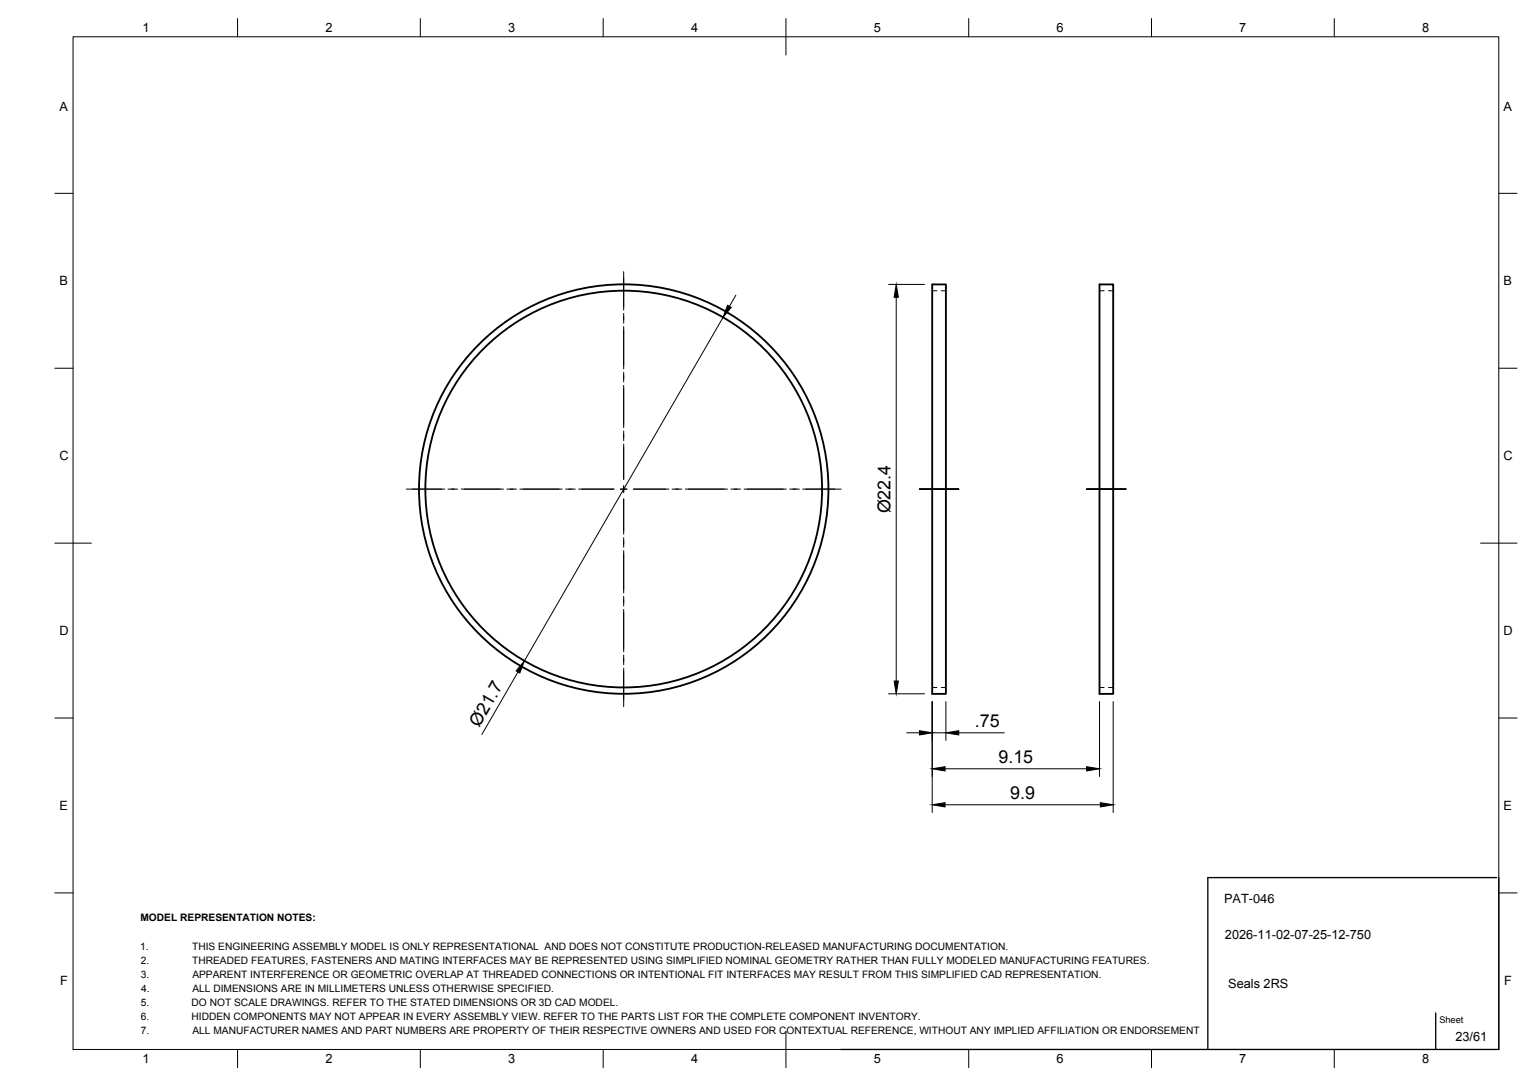
ISO-10303-21;
HEADER;
/* Generated by software containing ST-Developer
 * from STEP Tools, Inc. (www.steptools.com) 
 */

FILE_DESCRIPTION(
/* description */ ('Gear mesh backlash fixture'),
/* implementation_level */ '2;1');

FILE_NAME(
/* name */ 'Seals 2RS.step',
/* time_stamp */ '2026-10-28T03:26:00-07:00',
/* author */ (''),
/* organization */ (''),
/* preprocessor_version */ 'ST-DEVELOPER v20.2',
/* originating_system */ 'Autodesk Translation Framework v15.17.0.0',
/* authorisation */ '');

FILE_SCHEMA (('AUTOMOTIVE_DESIGN { 1 0 10303 214 3 1 1 }'));
ENDSEC;

DATA;
#10=MECHANICAL_DESIGN_GEOMETRIC_PRESENTATION_REPRESENTATION('',(#1038,#1039),#57900);
#932=SHAPE_REPRESENTATION_RELATIONSHIP('SRR','None',#58128,#982);
#982=ADVANCED_BREP_SHAPE_REPRESENTATION('',(#1103,#1104),#57861);
#1038=STYLED_ITEM('',(#58465),#1103);
#1039=STYLED_ITEM('',(#58465),#1104);
#1103=MANIFOLD_SOLID_BREP('Body1',#13598);
#1104=MANIFOLD_SOLID_BREP('Body2',#13599);
#1222=FACE_BOUND('',#2725,.T.);
#1223=FACE_BOUND('',#2728,.T.);
#1224=FACE_BOUND('',#2731,.T.);
#1225=FACE_BOUND('',#2734,.T.);
#1425=PLANE('',#14603);
#1426=PLANE('',#14608);
#1427=PLANE('',#14611);
#1428=PLANE('',#14616);
#1880=FACE_OUTER_BOUND('',#2724,.T.);
#1881=FACE_OUTER_BOUND('',#2726,.T.);
#1882=FACE_OUTER_BOUND('',#2727,.T.);
#1883=FACE_OUTER_BOUND('',#2729,.T.);
#1884=FACE_OUTER_BOUND('',#2730,.T.);
#1885=FACE_OUTER_BOUND('',#2732,.T.);
#1886=FACE_OUTER_BOUND('',#2733,.T.);
#1887=FACE_OUTER_BOUND('',#2735,.T.);
#2724=EDGE_LOOP('',(#9721));
#2725=EDGE_LOOP('',(#9722));
#2726=EDGE_LOOP('',(#9723,#9724,#9725,#9726));
#2727=EDGE_LOOP('',(#9727));
#2728=EDGE_LOOP('',(#9728));
#2729=EDGE_LOOP('',(#9729,#9730,#9731,#9732));
#2730=EDGE_LOOP('',(#9733));
#2731=EDGE_LOOP('',(#9734));
#2732=EDGE_LOOP('',(#9735,#9736,#9737,#9738));
#2733=EDGE_LOOP('',(#9739));
#2734=EDGE_LOOP('',(#9740));
#2735=EDGE_LOOP('',(#9741,#9742,#9743,#9744));
#3609=LINE('',#20541,#4498);
#3610=LINE('',#20546,#4499);
#3611=LINE('',#20555,#4500);
#3612=LINE('',#20560,#4501);
#4498=VECTOR('',#16602,1.119765);
#4499=VECTOR('',#16609,1.085235);
#4500=VECTOR('',#16620,1.119765);
#4501=VECTOR('',#16627,1.085235);
#5391=CIRCLE('',#14604,1.119765);
#5392=CIRCLE('',#14605,1.085235);
#5393=CIRCLE('',#14607,1.119765);
#5394=CIRCLE('',#14609,1.085235);
#5395=CIRCLE('',#14612,1.119765);
#5396=CIRCLE('',#14613,1.085235);
#5397=CIRCLE('',#14615,1.119765);
#5398=CIRCLE('',#14617,1.085235);
#6065=VERTEX_POINT('',#20534);
#6066=VERTEX_POINT('',#20536);
#6067=VERTEX_POINT('',#20539);
#6068=VERTEX_POINT('',#20543);
#6069=VERTEX_POINT('',#20548);
#6070=VERTEX_POINT('',#20550);
#6071=VERTEX_POINT('',#20553);
#6072=VERTEX_POINT('',#20557);
#7447=EDGE_CURVE('',#6065,#6065,#5391,.T.);
#7448=EDGE_CURVE('',#6066,#6066,#5392,.T.);
#7449=EDGE_CURVE('',#6067,#6067,#5393,.T.);
#7450=EDGE_CURVE('',#6067,#6065,#3609,.T.);
#7451=EDGE_CURVE('',#6068,#6068,#5394,.T.);
#7452=EDGE_CURVE('',#6068,#6066,#3610,.T.);
#7453=EDGE_CURVE('',#6069,#6069,#5395,.T.);
#7454=EDGE_CURVE('',#6070,#6070,#5396,.T.);
#7455=EDGE_CURVE('',#6071,#6071,#5397,.T.);
#7456=EDGE_CURVE('',#6071,#6069,#3611,.T.);
#7457=EDGE_CURVE('',#6072,#6072,#5398,.T.);
#7458=EDGE_CURVE('',#6072,#6070,#3612,.T.);
#9721=ORIENTED_EDGE('',*,*,#7447,.F.);
#9722=ORIENTED_EDGE('',*,*,#7448,.T.);
#9723=ORIENTED_EDGE('',*,*,#7449,.F.);
#9724=ORIENTED_EDGE('',*,*,#7450,.T.);
#9725=ORIENTED_EDGE('',*,*,#7447,.T.);
#9726=ORIENTED_EDGE('',*,*,#7450,.F.);
#9727=ORIENTED_EDGE('',*,*,#7449,.T.);
#9728=ORIENTED_EDGE('',*,*,#7451,.F.);
#9729=ORIENTED_EDGE('',*,*,#7451,.T.);
#9730=ORIENTED_EDGE('',*,*,#7452,.T.);
#9731=ORIENTED_EDGE('',*,*,#7448,.F.);
#9732=ORIENTED_EDGE('',*,*,#7452,.F.);
#9733=ORIENTED_EDGE('',*,*,#7453,.F.);
#9734=ORIENTED_EDGE('',*,*,#7454,.T.);
#9735=ORIENTED_EDGE('',*,*,#7455,.F.);
#9736=ORIENTED_EDGE('',*,*,#7456,.T.);
#9737=ORIENTED_EDGE('',*,*,#7453,.T.);
#9738=ORIENTED_EDGE('',*,*,#7456,.F.);
#9739=ORIENTED_EDGE('',*,*,#7455,.T.);
#9740=ORIENTED_EDGE('',*,*,#7457,.F.);
#9741=ORIENTED_EDGE('',*,*,#7457,.T.);
#9742=ORIENTED_EDGE('',*,*,#7458,.T.);
#9743=ORIENTED_EDGE('',*,*,#7454,.F.);
#9744=ORIENTED_EDGE('',*,*,#7458,.F.);
#12656=CYLINDRICAL_SURFACE('',#14606,1.119765);
#12657=CYLINDRICAL_SURFACE('',#14610,1.085235);
#12658=CYLINDRICAL_SURFACE('',#14614,1.119765);
#12659=CYLINDRICAL_SURFACE('',#14618,1.085235);
#12997=ADVANCED_FACE('',(#1880,#1222),#1425,.T.);
#12998=ADVANCED_FACE('',(#1881),#12656,.T.);
#12999=ADVANCED_FACE('',(#1882,#1223),#1426,.T.);
#13000=ADVANCED_FACE('',(#1883),#12657,.F.);
#13001=ADVANCED_FACE('',(#1884,#1224),#1427,.T.);
#13002=ADVANCED_FACE('',(#1885),#12658,.T.);
#13003=ADVANCED_FACE('',(#1886,#1225),#1428,.T.);
#13004=ADVANCED_FACE('',(#1887),#12659,.F.);
#13598=CLOSED_SHELL('',(#12997,#12998,#12999,#13000));
#13599=CLOSED_SHELL('',(#13001,#13002,#13003,#13004));
#14602=AXIS2_PLACEMENT_3D('',#20532,#16590,#16591);
#14603=AXIS2_PLACEMENT_3D('',#20533,#16592,#16593);
#14604=AXIS2_PLACEMENT_3D('',#20535,#16594,#16595);
#14605=AXIS2_PLACEMENT_3D('',#20537,#16596,#16597);
#14606=AXIS2_PLACEMENT_3D('',#20538,#16598,#16599);
#14607=AXIS2_PLACEMENT_3D('',#20540,#16600,#16601);
#14608=AXIS2_PLACEMENT_3D('',#20542,#16603,#16604);
#14609=AXIS2_PLACEMENT_3D('',#20544,#16605,#16606);
#14610=AXIS2_PLACEMENT_3D('',#20545,#16607,#16608);
#14611=AXIS2_PLACEMENT_3D('',#20547,#16610,#16611);
#14612=AXIS2_PLACEMENT_3D('',#20549,#16612,#16613);
#14613=AXIS2_PLACEMENT_3D('',#20551,#16614,#16615);
#14614=AXIS2_PLACEMENT_3D('',#20552,#16616,#16617);
#14615=AXIS2_PLACEMENT_3D('',#20554,#16618,#16619);
#14616=AXIS2_PLACEMENT_3D('',#20556,#16621,#16622);
#14617=AXIS2_PLACEMENT_3D('',#20558,#16623,#16624);
#14618=AXIS2_PLACEMENT_3D('',#20559,#16625,#16626);
#16590=DIRECTION('axis',(0.,0.,1.));
#16591=DIRECTION('refdir',(1.,0.,0.));
#16592=DIRECTION('center_axis',(0.,1.,0.));
#16593=DIRECTION('ref_axis',(0.,0.,1.));
#16594=DIRECTION('center_axis',(0.,-1.,0.));
#16595=DIRECTION('ref_axis',(1.,0.,0.));
#16596=DIRECTION('center_axis',(0.,-1.,0.));
#16597=DIRECTION('ref_axis',(1.,0.,0.));
#16598=DIRECTION('center_axis',(0.,-1.,0.));
#16599=DIRECTION('ref_axis',(1.,0.,0.));
#16600=DIRECTION('center_axis',(0.,-1.,0.));
#16601=DIRECTION('ref_axis',(1.,0.,0.));
#16602=DIRECTION('',(0.,1.,0.));
#16603=DIRECTION('center_axis',(0.,-1.,0.));
#16604=DIRECTION('ref_axis',(0.,0.,-1.));
#16605=DIRECTION('center_axis',(0.,-1.,0.));
#16606=DIRECTION('ref_axis',(1.,0.,0.));
#16607=DIRECTION('center_axis',(0.,-1.,0.));
#16608=DIRECTION('ref_axis',(1.,0.,0.));
#16609=DIRECTION('',(0.,1.,0.));
#16610=DIRECTION('center_axis',(0.,1.,0.));
#16611=DIRECTION('ref_axis',(0.,0.,1.));
#16612=DIRECTION('center_axis',(0.,-1.,0.));
#16613=DIRECTION('ref_axis',(1.,0.,0.));
#16614=DIRECTION('center_axis',(0.,-1.,0.));
#16615=DIRECTION('ref_axis',(1.,0.,0.));
#16616=DIRECTION('center_axis',(0.,-1.,0.));
#16617=DIRECTION('ref_axis',(1.,0.,0.));
#16618=DIRECTION('center_axis',(0.,-1.,0.));
#16619=DIRECTION('ref_axis',(1.,0.,0.));
#16620=DIRECTION('',(0.,1.,0.));
#16621=DIRECTION('center_axis',(0.,-1.,0.));
#16622=DIRECTION('ref_axis',(0.,0.,-1.));
#16623=DIRECTION('center_axis',(0.,-1.,0.));
#16624=DIRECTION('ref_axis',(1.,0.,0.));
#16625=DIRECTION('center_axis',(0.,-1.,0.));
#16626=DIRECTION('ref_axis',(1.,0.,0.));
#16627=DIRECTION('',(0.,1.,0.));
#20532=CARTESIAN_POINT('',(0.,0.,0.));
#20533=CARTESIAN_POINT('Origin',(1.119765,0.495,0.));
#20534=CARTESIAN_POINT('',(-1.119765,0.495,-1.37131662304724E-16));
#20535=CARTESIAN_POINT('Origin',(0.,0.495,0.));
#20536=CARTESIAN_POINT('',(-1.085235,0.495,-1.32902956907268E-16));
#20537=CARTESIAN_POINT('Origin',(0.,0.495,0.));
#20538=CARTESIAN_POINT('Origin',(0.,0.4575,0.));
#20539=CARTESIAN_POINT('',(-1.119765,0.42,-1.37131662304724E-16));
#20540=CARTESIAN_POINT('Origin',(0.,0.42,0.));
#20541=CARTESIAN_POINT('',(-1.119765,0.4575,-1.37131662304724E-16));
#20542=CARTESIAN_POINT('Origin',(1.085235,0.42,0.));
#20543=CARTESIAN_POINT('',(-1.085235,0.42,-1.32902956907268E-16));
#20544=CARTESIAN_POINT('Origin',(0.,0.42,0.));
#20545=CARTESIAN_POINT('Origin',(0.,0.4575,0.));
#20546=CARTESIAN_POINT('',(-1.085235,0.4575,-1.32902956907268E-16));
#20547=CARTESIAN_POINT('Origin',(1.119765,-0.42,0.));
#20548=CARTESIAN_POINT('',(-1.119765,-0.42,-1.37131662304724E-16));
#20549=CARTESIAN_POINT('Origin',(0.,-0.42,0.));
#20550=CARTESIAN_POINT('',(-1.085235,-0.42,-1.32902956907268E-16));
#20551=CARTESIAN_POINT('Origin',(0.,-0.42,0.));
#20552=CARTESIAN_POINT('Origin',(0.,-0.4575,0.));
#20553=CARTESIAN_POINT('',(-1.119765,-0.495,-1.37131662304724E-16));
#20554=CARTESIAN_POINT('Origin',(0.,-0.495,0.));
#20555=CARTESIAN_POINT('',(-1.119765,-0.4575,-1.37131662304724E-16));
#20556=CARTESIAN_POINT('Origin',(1.085235,-0.495,0.));
#20557=CARTESIAN_POINT('',(-1.085235,-0.495,-1.32902956907268E-16));
#20558=CARTESIAN_POINT('Origin',(0.,-0.495,0.));
#20559=CARTESIAN_POINT('Origin',(0.,-0.4575,0.));
#20560=CARTESIAN_POINT('',(-1.085235,-0.4575,-1.32902956907268E-16));
#57802=UNCERTAINTY_MEASURE_WITH_UNIT(LENGTH_MEASURE(0.001),#57901,
'DISTANCE_ACCURACY_VALUE',
'Maximum model space distance between geometric entities at asserted c
onnectivities');
#57841=UNCERTAINTY_MEASURE_WITH_UNIT(LENGTH_MEASURE(0.001),#57901,
'DISTANCE_ACCURACY_VALUE',
'Maximum model space distance between geometric entities at asserted c
onnectivities');
#57861=(
GEOMETRIC_REPRESENTATION_CONTEXT(3)
GLOBAL_UNCERTAINTY_ASSIGNED_CONTEXT((#57802))
GLOBAL_UNIT_ASSIGNED_CONTEXT((#57901,#57903,#57904))
REPRESENTATION_CONTEXT('','3D')
);
#57900=(
GEOMETRIC_REPRESENTATION_CONTEXT(3)
GLOBAL_UNCERTAINTY_ASSIGNED_CONTEXT((#57841))
GLOBAL_UNIT_ASSIGNED_CONTEXT((#57901,#57903,#57904))
REPRESENTATION_CONTEXT('','3D')
);
#57901=(
LENGTH_UNIT()
NAMED_UNIT(*)
SI_UNIT(.CENTI.,.METRE.)
);
#57903=(
NAMED_UNIT(*)
PLANE_ANGLE_UNIT()
SI_UNIT($,.RADIAN.)
);
#57904=(
NAMED_UNIT(*)
SI_UNIT($,.STERADIAN.)
SOLID_ANGLE_UNIT()
);
#57924=SHAPE_DEFINITION_REPRESENTATION(#57982,#58128);
#57982=PRODUCT_DEFINITION_SHAPE('',$,#58187);
#58128=SHAPE_REPRESENTATION('',(#14602),#57861);
#58167=PRODUCT_DEFINITION_CONTEXT('part definition',#58343,'design');
#58187=PRODUCT_DEFINITION('Seals 2RS','Seals 2RS',#58245,#58167);
#58245=PRODUCT_DEFINITION_FORMATION('',$,#58364);
#58343=APPLICATION_CONTEXT(
'Core Data for Automotive Mechanical Design Process');
#58344=PRODUCT_CONTEXT('part definition',#58343,'mechanical');
#58364=PRODUCT('Seals 2RS','Seals 2RS','Seals 2RS',(#58344));
#58459=COLOUR_RGB('Grey',0.48,0.52,0.57);
#58460=FILL_AREA_STYLE_COLOUR('',#58459);
#58461=FILL_AREA_STYLE('',(#58460));
#58462=SURFACE_STYLE_FILL_AREA(#58461);
#58463=SURFACE_SIDE_STYLE('',(#58462));
#58464=SURFACE_STYLE_USAGE(.BOTH.,#58463);
#58465=PRESENTATION_STYLE_ASSIGNMENT((#58464));
ENDSEC;
END-ISO-10303-21;
